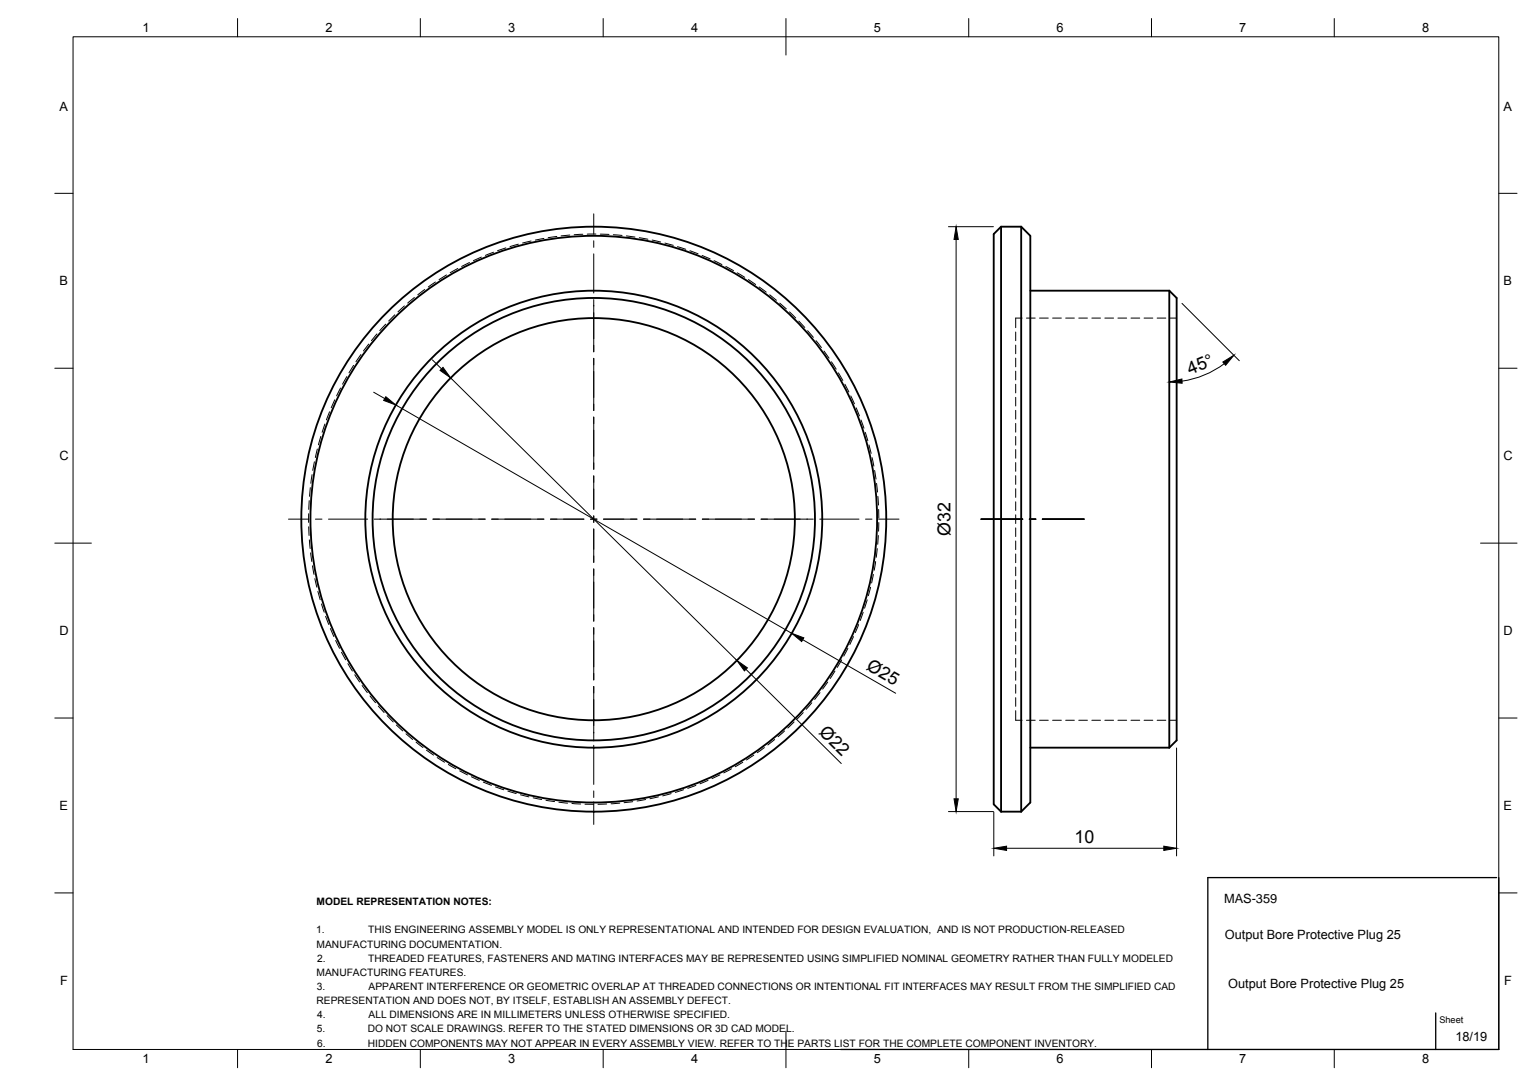
ISO-10303-21;
HEADER;
/* Generated by software containing ST-Developer
 * from STEP Tools, Inc. (www.steptools.com) 
 */

FILE_DESCRIPTION(
/* description */ (''),
/* implementation_level */ '2;1');

FILE_NAME(
/* name */ 'Output Bore Protective Plug 25.step',
/* time_stamp */ '2026-10-15T14:25:16-07:00',
/* author */ (''),
/* organization */ (''),
/* preprocessor_version */ 'ST-DEVELOPER v20.2',
/* originating_system */ 'Autodesk Translation Framework v15.15.0.0',
/* authorisation */ '');

FILE_SCHEMA (('AUTOMOTIVE_DESIGN { 1 0 10303 214 3 1 1 }'));
ENDSEC;

DATA;
#10=MECHANICAL_DESIGN_GEOMETRIC_PRESENTATION_REPRESENTATION('',(#340),#86429);
#304=SHAPE_REPRESENTATION_RELATIONSHIP('SRR','None',#86519,#322);
#322=ADVANCED_BREP_SHAPE_REPRESENTATION('',(#358),#86428);
#340=STYLED_ITEM('',(#86611),#358);
#358=MANIFOLD_SOLID_BREP('Body1',#15630);
#1348=CONICAL_SURFACE('',#17243,1.23,0.785398163397448);
#1349=CONICAL_SURFACE('',#17249,1.575,0.785398163397449);
#1350=CONICAL_SURFACE('',#17253,1.58,0.785398163397449);
#1599=CYLINDRICAL_SURFACE('',#17238,1.1);
#1600=CYLINDRICAL_SURFACE('',#17245,1.25);
#1601=CYLINDRICAL_SURFACE('',#17251,1.6);
#1752=FACE_BOUND('',#4271,.T.);
#1753=FACE_BOUND('',#4275,.T.);
#2376=CIRCLE('',#17239,1.1);
#2377=CIRCLE('',#17240,1.1);
#2378=CIRCLE('',#17242,1.21);
#2379=CIRCLE('',#17244,1.25);
#2380=CIRCLE('',#17246,1.25);
#2381=CIRCLE('',#17248,1.55);
#2382=CIRCLE('',#17250,1.6);
#2383=CIRCLE('',#17252,1.6);
#2384=CIRCLE('',#17254,1.56);
#3247=FACE_OUTER_BOUND('',#4269,.T.);
#3248=FACE_OUTER_BOUND('',#4270,.T.);
#3249=FACE_OUTER_BOUND('',#4272,.T.);
#3250=FACE_OUTER_BOUND('',#4273,.T.);
#3251=FACE_OUTER_BOUND('',#4274,.T.);
#3252=FACE_OUTER_BOUND('',#4276,.T.);
#3253=FACE_OUTER_BOUND('',#4277,.T.);
#3254=FACE_OUTER_BOUND('',#4278,.T.);
#3255=FACE_OUTER_BOUND('',#4279,.T.);
#3256=FACE_OUTER_BOUND('',#4280,.T.);
#4269=EDGE_LOOP('',(#14429,#14430,#14431,#14432));
#4270=EDGE_LOOP('',(#14433));
#4271=EDGE_LOOP('',(#14434));
#4272=EDGE_LOOP('',(#14435,#14436,#14437,#14438));
#4273=EDGE_LOOP('',(#14439,#14440,#14441,#14442));
#4274=EDGE_LOOP('',(#14443));
#4275=EDGE_LOOP('',(#14444));
#4276=EDGE_LOOP('',(#14445,#14446,#14447,#14448));
#4277=EDGE_LOOP('',(#14449,#14450,#14451,#14452));
#4278=EDGE_LOOP('',(#14453,#14454,#14455,#14456));
#4279=EDGE_LOOP('',(#14457));
#4280=EDGE_LOOP('',(#14458));
#5135=LINE('',#86331,#5995);
#5136=LINE('',#86339,#5996);
#5137=LINE('',#86343,#5997);
#5138=LINE('',#86350,#5998);
#5139=LINE('',#86354,#5999);
#5140=LINE('',#86357,#6000);
#5995=VECTOR('',#20960,1.1);
#5996=VECTOR('',#20971,1.23);
#5997=VECTOR('',#20976,1.25);
#5998=VECTOR('',#20985,1.575);
#5999=VECTOR('',#20990,1.6);
#6000=VECTOR('',#20993,1.58);
#7538=VERTEX_POINT('',#86328);
#7539=VERTEX_POINT('',#86330);
#7540=VERTEX_POINT('',#86334);
#7541=VERTEX_POINT('',#86337);
#7542=VERTEX_POINT('',#86341);
#7543=VERTEX_POINT('',#86345);
#7544=VERTEX_POINT('',#86348);
#7545=VERTEX_POINT('',#86352);
#7546=VERTEX_POINT('',#86356);
#9836=EDGE_CURVE('',#7538,#7538,#2376,.T.);
#9837=EDGE_CURVE('',#7538,#7539,#5135,.T.);
#9838=EDGE_CURVE('',#7539,#7539,#2377,.T.);
#9839=EDGE_CURVE('',#7540,#7540,#2378,.T.);
#9840=EDGE_CURVE('',#7541,#7541,#2379,.T.);
#9841=EDGE_CURVE('',#7541,#7540,#5136,.T.);
#9842=EDGE_CURVE('',#7542,#7542,#2380,.T.);
#9843=EDGE_CURVE('',#7542,#7541,#5137,.T.);
#9844=EDGE_CURVE('',#7543,#7543,#2381,.T.);
#9845=EDGE_CURVE('',#7544,#7544,#2382,.T.);
#9846=EDGE_CURVE('',#7544,#7543,#5138,.T.);
#9847=EDGE_CURVE('',#7545,#7545,#2383,.T.);
#9848=EDGE_CURVE('',#7545,#7544,#5139,.T.);
#9849=EDGE_CURVE('',#7545,#7546,#5140,.T.);
#9850=EDGE_CURVE('',#7546,#7546,#2384,.T.);
#14429=ORIENTED_EDGE('',*,*,#9836,.F.);
#14430=ORIENTED_EDGE('',*,*,#9837,.T.);
#14431=ORIENTED_EDGE('',*,*,#9838,.T.);
#14432=ORIENTED_EDGE('',*,*,#9837,.F.);
#14433=ORIENTED_EDGE('',*,*,#9839,.F.);
#14434=ORIENTED_EDGE('',*,*,#9836,.T.);
#14435=ORIENTED_EDGE('',*,*,#9840,.F.);
#14436=ORIENTED_EDGE('',*,*,#9841,.T.);
#14437=ORIENTED_EDGE('',*,*,#9839,.T.);
#14438=ORIENTED_EDGE('',*,*,#9841,.F.);
#14439=ORIENTED_EDGE('',*,*,#9842,.F.);
#14440=ORIENTED_EDGE('',*,*,#9843,.T.);
#14441=ORIENTED_EDGE('',*,*,#9840,.T.);
#14442=ORIENTED_EDGE('',*,*,#9843,.F.);
#14443=ORIENTED_EDGE('',*,*,#9844,.F.);
#14444=ORIENTED_EDGE('',*,*,#9842,.T.);
#14445=ORIENTED_EDGE('',*,*,#9845,.F.);
#14446=ORIENTED_EDGE('',*,*,#9846,.T.);
#14447=ORIENTED_EDGE('',*,*,#9844,.T.);
#14448=ORIENTED_EDGE('',*,*,#9846,.F.);
#14449=ORIENTED_EDGE('',*,*,#9847,.F.);
#14450=ORIENTED_EDGE('',*,*,#9848,.T.);
#14451=ORIENTED_EDGE('',*,*,#9845,.T.);
#14452=ORIENTED_EDGE('',*,*,#9848,.F.);
#14453=ORIENTED_EDGE('',*,*,#9847,.T.);
#14454=ORIENTED_EDGE('',*,*,#9849,.T.);
#14455=ORIENTED_EDGE('',*,*,#9850,.F.);
#14456=ORIENTED_EDGE('',*,*,#9849,.F.);
#14457=ORIENTED_EDGE('',*,*,#9850,.T.);
#14458=ORIENTED_EDGE('',*,*,#9838,.F.);
#14737=PLANE('',#17241);
#14738=PLANE('',#17247);
#14739=PLANE('',#17255);
#14740=PLANE('',#17256);
#15603=ADVANCED_FACE('',(#3247),#1599,.F.);
#15604=ADVANCED_FACE('',(#3248,#1752),#14737,.T.);
#15605=ADVANCED_FACE('',(#3249),#1348,.T.);
#15606=ADVANCED_FACE('',(#3250),#1600,.T.);
#15607=ADVANCED_FACE('',(#3251,#1753),#14738,.T.);
#15608=ADVANCED_FACE('',(#3252),#1349,.T.);
#15609=ADVANCED_FACE('',(#3253),#1601,.T.);
#15610=ADVANCED_FACE('',(#3254),#1350,.T.);
#15611=ADVANCED_FACE('',(#3255),#14739,.T.);
#15612=ADVANCED_FACE('',(#3256),#14740,.T.);
#15630=CLOSED_SHELL('',(#15603,#15604,#15605,#15606,#15607,#15608,#15609,
#15610,#15611,#15612));
#17237=AXIS2_PLACEMENT_3D('',#86326,#20954,#20955);
#17238=AXIS2_PLACEMENT_3D('',#86327,#20956,#20957);
#17239=AXIS2_PLACEMENT_3D('',#86329,#20958,#20959);
#17240=AXIS2_PLACEMENT_3D('',#86332,#20961,#20962);
#17241=AXIS2_PLACEMENT_3D('',#86333,#20963,#20964);
#17242=AXIS2_PLACEMENT_3D('',#86335,#20965,#20966);
#17243=AXIS2_PLACEMENT_3D('',#86336,#20967,#20968);
#17244=AXIS2_PLACEMENT_3D('',#86338,#20969,#20970);
#17245=AXIS2_PLACEMENT_3D('',#86340,#20972,#20973);
#17246=AXIS2_PLACEMENT_3D('',#86342,#20974,#20975);
#17247=AXIS2_PLACEMENT_3D('',#86344,#20977,#20978);
#17248=AXIS2_PLACEMENT_3D('',#86346,#20979,#20980);
#17249=AXIS2_PLACEMENT_3D('',#86347,#20981,#20982);
#17250=AXIS2_PLACEMENT_3D('',#86349,#20983,#20984);
#17251=AXIS2_PLACEMENT_3D('',#86351,#20986,#20987);
#17252=AXIS2_PLACEMENT_3D('',#86353,#20988,#20989);
#17253=AXIS2_PLACEMENT_3D('',#86355,#20991,#20992);
#17254=AXIS2_PLACEMENT_3D('',#86358,#20994,#20995);
#17255=AXIS2_PLACEMENT_3D('',#86359,#20996,#20997);
#17256=AXIS2_PLACEMENT_3D('',#86360,#20998,#20999);
#20954=DIRECTION('axis',(0.,0.,1.));
#20955=DIRECTION('refdir',(1.,0.,0.));
#20956=DIRECTION('center_axis',(0.,0.,1.));
#20957=DIRECTION('ref_axis',(1.,0.,0.));
#20958=DIRECTION('center_axis',(0.,0.,1.));
#20959=DIRECTION('ref_axis',(1.,0.,0.));
#20960=DIRECTION('',(0.,0.,1.));
#20961=DIRECTION('center_axis',(0.,0.,1.));
#20962=DIRECTION('ref_axis',(1.,0.,0.));
#20963=DIRECTION('center_axis',(0.,0.,-1.));
#20964=DIRECTION('ref_axis',(-1.,0.,0.));
#20965=DIRECTION('center_axis',(0.,0.,1.));
#20966=DIRECTION('ref_axis',(1.,0.,0.));
#20967=DIRECTION('center_axis',(0.,0.,1.));
#20968=DIRECTION('ref_axis',(1.,0.,0.));
#20969=DIRECTION('center_axis',(0.,0.,1.));
#20970=DIRECTION('ref_axis',(1.,0.,0.));
#20971=DIRECTION('',(0.707106781186547,8.65956056235493E-17,-0.707106781186548));
#20972=DIRECTION('center_axis',(0.,0.,1.));
#20973=DIRECTION('ref_axis',(1.,0.,0.));
#20974=DIRECTION('center_axis',(0.,0.,1.));
#20975=DIRECTION('ref_axis',(1.,0.,0.));
#20976=DIRECTION('',(0.,0.,-1.));
#20977=DIRECTION('center_axis',(0.,0.,-1.));
#20978=DIRECTION('ref_axis',(-1.,0.,0.));
#20979=DIRECTION('center_axis',(0.,0.,1.));
#20980=DIRECTION('ref_axis',(1.,0.,0.));
#20981=DIRECTION('center_axis',(0.,0.,1.));
#20982=DIRECTION('ref_axis',(1.,0.,0.));
#20983=DIRECTION('center_axis',(0.,0.,1.));
#20984=DIRECTION('ref_axis',(1.,0.,0.));
#20985=DIRECTION('',(0.707106781186548,8.65956056235494E-17,-0.707106781186547));
#20986=DIRECTION('center_axis',(0.,0.,1.));
#20987=DIRECTION('ref_axis',(1.,0.,0.));
#20988=DIRECTION('center_axis',(0.,0.,1.));
#20989=DIRECTION('ref_axis',(1.,0.,0.));
#20990=DIRECTION('',(0.,0.,-1.));
#20991=DIRECTION('center_axis',(0.,0.,-1.));
#20992=DIRECTION('ref_axis',(1.,0.,0.));
#20993=DIRECTION('',(0.707106781186548,-8.65956056235494E-17,0.707106781186547));
#20994=DIRECTION('center_axis',(0.,0.,1.));
#20995=DIRECTION('ref_axis',(1.,0.,0.));
#20996=DIRECTION('center_axis',(0.,0.,1.));
#20997=DIRECTION('ref_axis',(1.,0.,0.));
#20998=DIRECTION('center_axis',(0.,0.,-1.));
#20999=DIRECTION('ref_axis',(-1.,0.,0.));
#86326=CARTESIAN_POINT('',(0.,0.,0.));
#86327=CARTESIAN_POINT('Origin',(0.,0.,-0.36));
#86328=CARTESIAN_POINT('',(-1.1,-1.34711147906209E-16,-0.8));
#86329=CARTESIAN_POINT('Origin',(0.,0.,-0.8));
#86330=CARTESIAN_POINT('',(-1.1,-1.34711147906209E-16,0.08));
#86331=CARTESIAN_POINT('',(-1.1,-1.34711147906209E-16,-0.36));
#86332=CARTESIAN_POINT('Origin',(0.,0.,0.08));
#86333=CARTESIAN_POINT('Origin',(1.21,0.,-0.8));
#86334=CARTESIAN_POINT('',(-1.21,-1.4818226269683E-16,-0.8));
#86335=CARTESIAN_POINT('Origin',(0.,0.,-0.8));
#86336=CARTESIAN_POINT('Origin',(0.,0.,-0.78));
#86337=CARTESIAN_POINT('',(-1.25,-1.53080849893419E-16,-0.76));
#86338=CARTESIAN_POINT('Origin',(0.,0.,-0.76));
#86339=CARTESIAN_POINT('',(-1.23,-1.50631556295124E-16,-0.78));
#86340=CARTESIAN_POINT('Origin',(0.,0.,-0.38));
#86341=CARTESIAN_POINT('',(-1.25,-1.53080849893419E-16,0.));
#86342=CARTESIAN_POINT('Origin',(0.,0.,0.));
#86343=CARTESIAN_POINT('',(-1.25,-1.53080849893419E-16,-0.38));
#86344=CARTESIAN_POINT('Origin',(1.55,0.,0.));
#86345=CARTESIAN_POINT('',(-1.55,-1.8982025386784E-16,-7.97972798949331E-17));
#86346=CARTESIAN_POINT('Origin',(0.,0.,0.));
#86347=CARTESIAN_POINT('Origin',(0.,0.,0.025));
#86348=CARTESIAN_POINT('',(-1.6,-1.95943487863577E-16,0.0499999999999999));
#86349=CARTESIAN_POINT('Origin',(0.,0.,0.05));
#86350=CARTESIAN_POINT('',(-1.575,-1.92881870865708E-16,0.025));
#86351=CARTESIAN_POINT('Origin',(0.,0.,0.105));
#86352=CARTESIAN_POINT('',(-1.6,-1.95943487863577E-16,0.16));
#86353=CARTESIAN_POINT('Origin',(0.,0.,0.16));
#86354=CARTESIAN_POINT('',(-1.6,-1.95943487863577E-16,0.105));
#86355=CARTESIAN_POINT('Origin',(0.,0.,0.18));
#86356=CARTESIAN_POINT('',(-1.56,-1.91044900666987E-16,0.2));
#86357=CARTESIAN_POINT('',(-1.58,1.93494194265282E-16,0.18));
#86358=CARTESIAN_POINT('Origin',(0.,0.,0.2));
#86359=CARTESIAN_POINT('Origin',(0.,0.,0.2));
#86360=CARTESIAN_POINT('Origin',(1.1,0.,0.08));
#86408=UNCERTAINTY_MEASURE_WITH_UNIT(LENGTH_MEASURE(0.001),#86430,
'DISTANCE_ACCURACY_VALUE',
'Maximum model space distance between geometric entities at asserted c
onnectivities');
#86409=UNCERTAINTY_MEASURE_WITH_UNIT(LENGTH_MEASURE(0.001),#86430,
'DISTANCE_ACCURACY_VALUE',
'Maximum model space distance between geometric entities at asserted c
onnectivities');
#86428=(
GEOMETRIC_REPRESENTATION_CONTEXT(3)
GLOBAL_UNCERTAINTY_ASSIGNED_CONTEXT((#86408))
GLOBAL_UNIT_ASSIGNED_CONTEXT((#86430,#86432,#86433))
REPRESENTATION_CONTEXT('','3D')
);
#86429=(
GEOMETRIC_REPRESENTATION_CONTEXT(3)
GLOBAL_UNCERTAINTY_ASSIGNED_CONTEXT((#86409))
GLOBAL_UNIT_ASSIGNED_CONTEXT((#86430,#86432,#86433))
REPRESENTATION_CONTEXT('','3D')
);
#86430=(
LENGTH_UNIT()
NAMED_UNIT(*)
SI_UNIT(.CENTI.,.METRE.)
);
#86432=(
NAMED_UNIT(*)
PLANE_ANGLE_UNIT()
SI_UNIT($,.RADIAN.)
);
#86433=(
NAMED_UNIT(*)
SI_UNIT($,.STERADIAN.)
SOLID_ANGLE_UNIT()
);
#86452=SHAPE_DEFINITION_REPRESENTATION(#86471,#86519);
#86471=PRODUCT_DEFINITION_SHAPE('',$,#86539);
#86519=SHAPE_REPRESENTATION('',(#17237),#86428);
#86520=PRODUCT_DEFINITION_CONTEXT('part definition',#86579,'design');
#86539=PRODUCT_DEFINITION('Output Bore Protective Plug 25',
'Output Bore Protective Plug 25',#86558,#86520);
#86558=PRODUCT_DEFINITION_FORMATION('',$,#86599);
#86579=APPLICATION_CONTEXT(
'Core Data for Automotive Mechanical Design Process');
#86580=PRODUCT_CONTEXT('part definition',#86579,'mechanical');
#86599=PRODUCT('Output Bore Protective Plug 25',
'Output Bore Protective Plug 25',$,(#86580));
#86611=PRESENTATION_STYLE_ASSIGNMENT((#86629));
#86629=SURFACE_STYLE_USAGE(.BOTH.,#86647);
#86647=SURFACE_SIDE_STYLE('',(#86665));
#86665=SURFACE_STYLE_FILL_AREA(#86683);
#86683=FILL_AREA_STYLE('Opaque(240,172,28)',(#86701));
#86701=FILL_AREA_STYLE_COLOUR('Opaque(240,172,28)',#86719);
#86719=COLOUR_RGB('Opaque(240,172,28)', 0.72549020, 0.75294118, 0.79215686);
ENDSEC;
END-ISO-10303-21;
